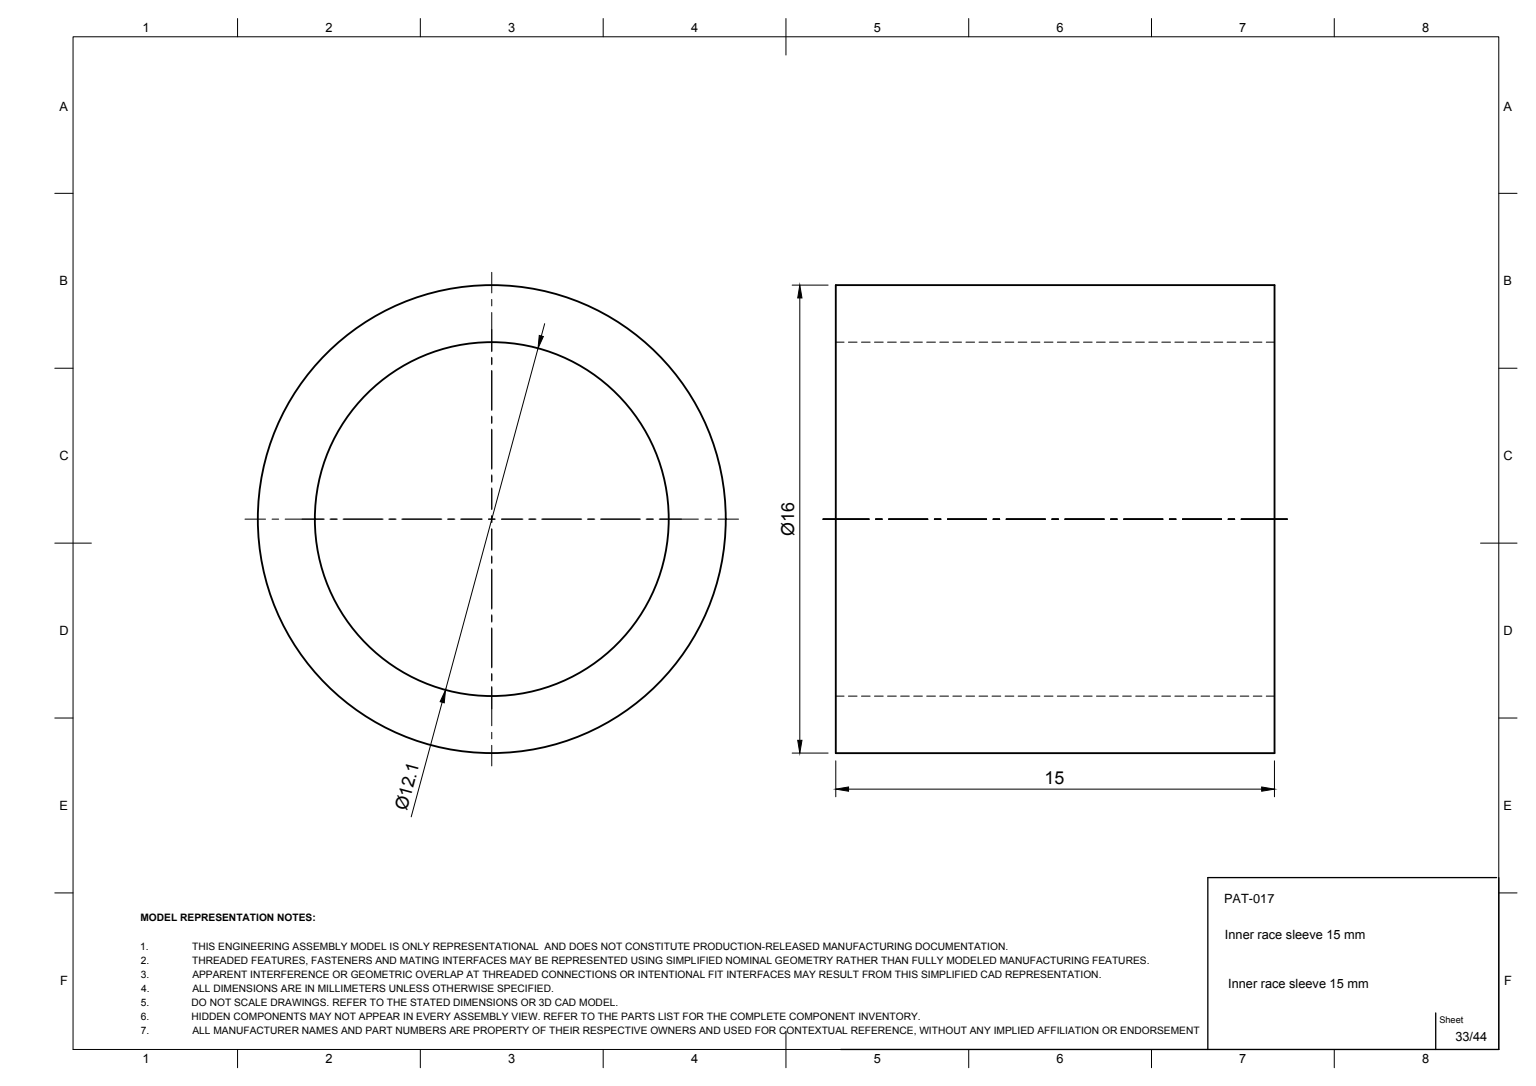
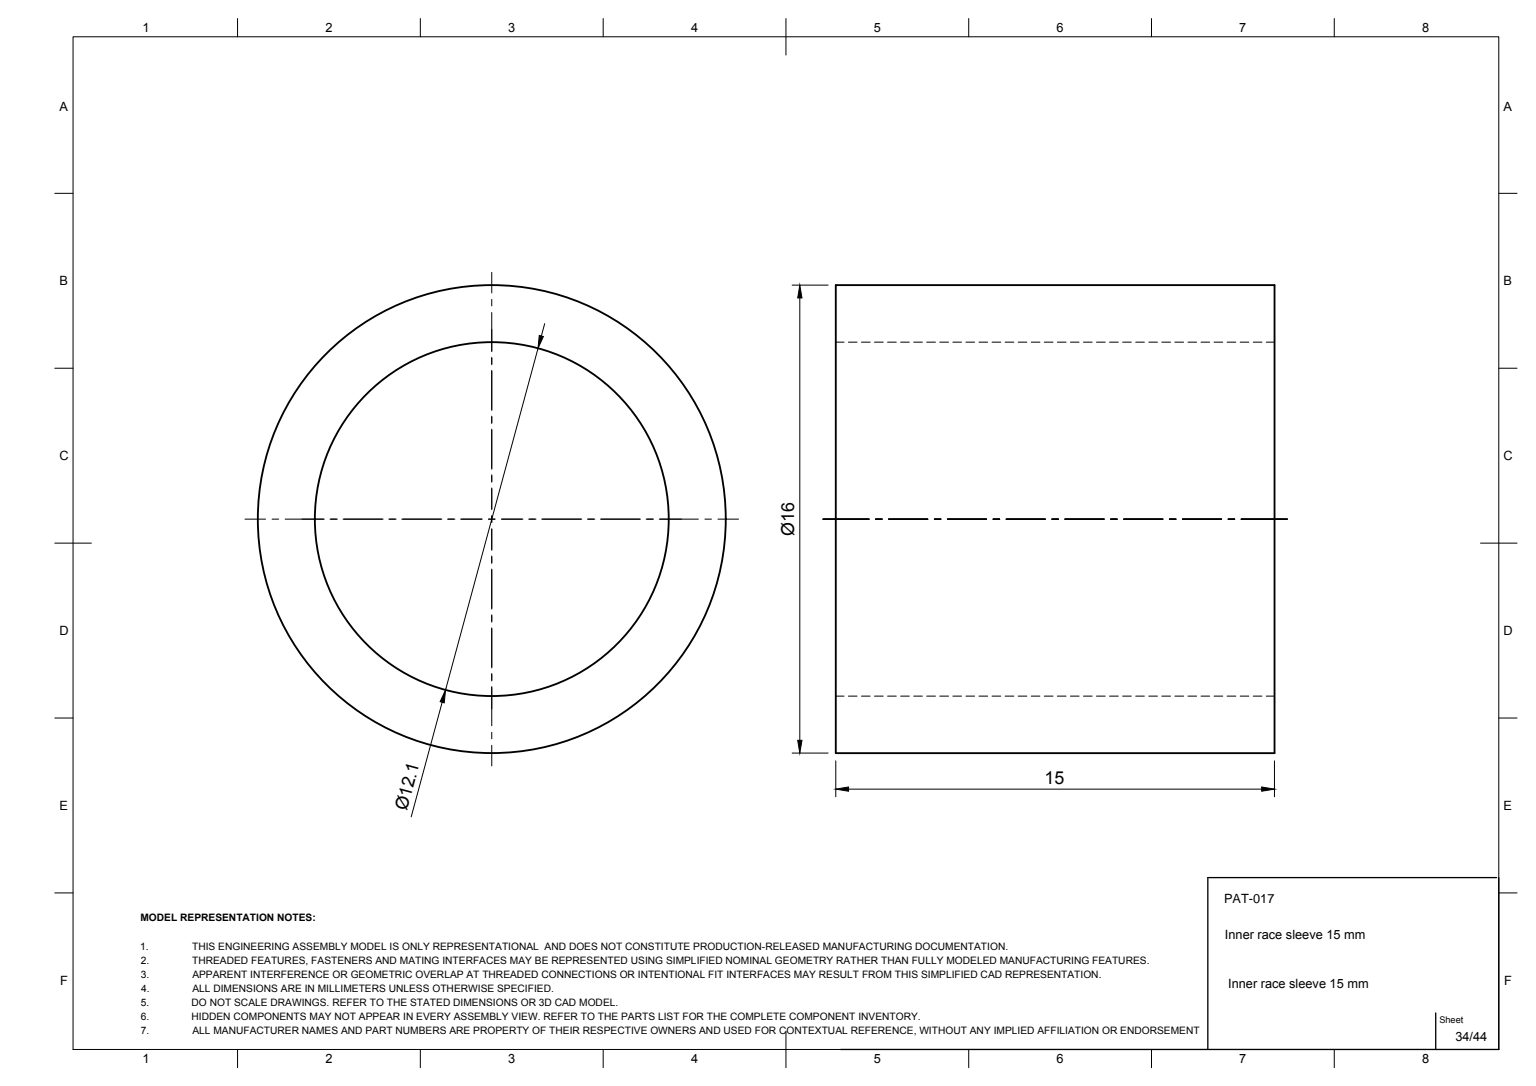
ISO-10303-21;
HEADER;
/* Generated by software containing ST-Developer
 * from STEP Tools, Inc. (www.steptools.com) 
 */

FILE_DESCRIPTION(
/* description */ ('Cam-and-follower valve demonstrator'),
/* implementation_level */ '2;1');

FILE_NAME(
/* name */ 'Inner race sleeve 15 mm.step',
/* time_stamp */ '2026-10-28T03:25:17-07:00',
/* author */ (''),
/* organization */ (''),
/* preprocessor_version */ 'ST-DEVELOPER v20.2',
/* originating_system */ 'Autodesk Translation Framework v15.17.0.0',
/* authorisation */ '');

FILE_SCHEMA (('AUTOMOTIVE_DESIGN { 1 0 10303 214 3 1 1 }'));
ENDSEC;

DATA;
#10=MECHANICAL_DESIGN_GEOMETRIC_PRESENTATION_REPRESENTATION('',(#443),#12896);
#364=SHAPE_REPRESENTATION_RELATIONSHIP('SRR','None',#13083,#400);
#400=ADVANCED_BREP_SHAPE_REPRESENTATION('',(#484),#12883);
#443=STYLED_ITEM('',(#13330),#484);
#484=MANIFOLD_SOLID_BREP('Body1',#6212);
#634=FACE_BOUND('',#1883,.T.);
#635=FACE_BOUND('',#1885,.T.);
#915=CIRCLE('',#7193,0.605);
#916=CIRCLE('',#7194,0.605);
#917=CIRCLE('',#7196,0.8);
#918=CIRCLE('',#7197,0.8);
#1069=CYLINDRICAL_SURFACE('',#7192,0.605);
#1070=CYLINDRICAL_SURFACE('',#7195,0.8);
#1373=FACE_OUTER_BOUND('',#1880,.T.);
#1374=FACE_OUTER_BOUND('',#1881,.T.);
#1375=FACE_OUTER_BOUND('',#1882,.T.);
#1376=FACE_OUTER_BOUND('',#1884,.T.);
#1880=EDGE_LOOP('',(#5263,#5264,#5265,#5266));
#1881=EDGE_LOOP('',(#5267,#5268,#5269,#5270));
#1882=EDGE_LOOP('',(#5271));
#1883=EDGE_LOOP('',(#5272));
#1884=EDGE_LOOP('',(#5273));
#1885=EDGE_LOOP('',(#5274));
#2308=LINE('',#12374,#2730);
#2309=LINE('',#12380,#2731);
#2730=VECTOR('',#8871,0.605);
#2731=VECTOR('',#8878,0.8);
#3234=VERTEX_POINT('',#12371);
#3235=VERTEX_POINT('',#12373);
#3236=VERTEX_POINT('',#12377);
#3237=VERTEX_POINT('',#12379);
#3928=EDGE_CURVE('',#3234,#3234,#915,.T.);
#3929=EDGE_CURVE('',#3234,#3235,#2308,.T.);
#3930=EDGE_CURVE('',#3235,#3235,#916,.T.);
#3931=EDGE_CURVE('',#3236,#3236,#917,.T.);
#3932=EDGE_CURVE('',#3236,#3237,#2309,.T.);
#3933=EDGE_CURVE('',#3237,#3237,#918,.T.);
#5263=ORIENTED_EDGE('',*,*,#3928,.F.);
#5264=ORIENTED_EDGE('',*,*,#3929,.T.);
#5265=ORIENTED_EDGE('',*,*,#3930,.T.);
#5266=ORIENTED_EDGE('',*,*,#3929,.F.);
#5267=ORIENTED_EDGE('',*,*,#3931,.F.);
#5268=ORIENTED_EDGE('',*,*,#3932,.T.);
#5269=ORIENTED_EDGE('',*,*,#3933,.T.);
#5270=ORIENTED_EDGE('',*,*,#3932,.F.);
#5271=ORIENTED_EDGE('',*,*,#3931,.T.);
#5272=ORIENTED_EDGE('',*,*,#3928,.T.);
#5273=ORIENTED_EDGE('',*,*,#3933,.F.);
#5274=ORIENTED_EDGE('',*,*,#3930,.F.);
#5751=PLANE('',#7198);
#5752=PLANE('',#7199);
#6089=ADVANCED_FACE('',(#1373),#1069,.F.);
#6090=ADVANCED_FACE('',(#1374),#1070,.T.);
#6091=ADVANCED_FACE('',(#1375,#634),#5751,.T.);
#6092=ADVANCED_FACE('',(#1376,#635),#5752,.F.);
#6212=CLOSED_SHELL('',(#6089,#6090,#6091,#6092));
#7191=AXIS2_PLACEMENT_3D('',#12369,#8865,#8866);
#7192=AXIS2_PLACEMENT_3D('',#12370,#8867,#8868);
#7193=AXIS2_PLACEMENT_3D('',#12372,#8869,#8870);
#7194=AXIS2_PLACEMENT_3D('',#12375,#8872,#8873);
#7195=AXIS2_PLACEMENT_3D('',#12376,#8874,#8875);
#7196=AXIS2_PLACEMENT_3D('',#12378,#8876,#8877);
#7197=AXIS2_PLACEMENT_3D('',#12381,#8879,#8880);
#7198=AXIS2_PLACEMENT_3D('',#12382,#8881,#8882);
#7199=AXIS2_PLACEMENT_3D('',#12383,#8883,#8884);
#8865=DIRECTION('axis',(0.,0.,1.));
#8866=DIRECTION('refdir',(1.,0.,0.));
#8867=DIRECTION('center_axis',(0.,1.,0.));
#8868=DIRECTION('ref_axis',(1.,0.,0.));
#8869=DIRECTION('center_axis',(0.,-1.,0.));
#8870=DIRECTION('ref_axis',(1.,0.,0.));
#8871=DIRECTION('',(0.,-1.,0.));
#8872=DIRECTION('center_axis',(0.,-1.,0.));
#8873=DIRECTION('ref_axis',(1.,0.,0.));
#8874=DIRECTION('center_axis',(0.,1.,0.));
#8875=DIRECTION('ref_axis',(1.,0.,0.));
#8876=DIRECTION('center_axis',(0.,1.,0.));
#8877=DIRECTION('ref_axis',(1.,0.,0.));
#8878=DIRECTION('',(0.,-1.,0.));
#8879=DIRECTION('center_axis',(0.,1.,0.));
#8880=DIRECTION('ref_axis',(1.,0.,0.));
#8881=DIRECTION('center_axis',(0.,1.,0.));
#8882=DIRECTION('ref_axis',(1.,0.,0.));
#8883=DIRECTION('center_axis',(0.,1.,0.));
#8884=DIRECTION('ref_axis',(1.,0.,0.));
#12369=CARTESIAN_POINT('',(0.,0.,0.));
#12370=CARTESIAN_POINT('Origin',(0.,-4.5,4.));
#12371=CARTESIAN_POINT('',(-0.605,-3.,4.));
#12372=CARTESIAN_POINT('Origin',(0.,-3.,4.));
#12373=CARTESIAN_POINT('',(-0.605,-4.5,4.));
#12374=CARTESIAN_POINT('',(-0.605,-4.5,4.));
#12375=CARTESIAN_POINT('Origin',(0.,-4.5,4.));
#12376=CARTESIAN_POINT('Origin',(0.,-4.5,4.));
#12377=CARTESIAN_POINT('',(-0.8,-3.,4.));
#12378=CARTESIAN_POINT('Origin',(0.,-3.,4.));
#12379=CARTESIAN_POINT('',(-0.8,-4.5,4.));
#12380=CARTESIAN_POINT('',(-0.8,-4.5,4.));
#12381=CARTESIAN_POINT('Origin',(0.,-4.5,4.));
#12382=CARTESIAN_POINT('Origin',(0.,-3.,4.));
#12383=CARTESIAN_POINT('Origin',(0.,-4.5,4.));
#12840=UNCERTAINTY_MEASURE_WITH_UNIT(LENGTH_MEASURE(0.001),#12897,
'DISTANCE_ACCURACY_VALUE',
'Maximum model space distance between geometric entities at asserted c
onnectivities');
#12853=UNCERTAINTY_MEASURE_WITH_UNIT(LENGTH_MEASURE(0.001),#12897,
'DISTANCE_ACCURACY_VALUE',
'Maximum model space distance between geometric entities at asserted c
onnectivities');
#12883=(
GEOMETRIC_REPRESENTATION_CONTEXT(3)
GLOBAL_UNCERTAINTY_ASSIGNED_CONTEXT((#12840))
GLOBAL_UNIT_ASSIGNED_CONTEXT((#12897,#12899,#12900))
REPRESENTATION_CONTEXT('','3D')
);
#12896=(
GEOMETRIC_REPRESENTATION_CONTEXT(3)
GLOBAL_UNCERTAINTY_ASSIGNED_CONTEXT((#12853))
GLOBAL_UNIT_ASSIGNED_CONTEXT((#12897,#12899,#12900))
REPRESENTATION_CONTEXT('','3D')
);
#12897=(
LENGTH_UNIT()
NAMED_UNIT(*)
SI_UNIT(.CENTI.,.METRE.)
);
#12899=(
NAMED_UNIT(*)
PLANE_ANGLE_UNIT()
SI_UNIT($,.RADIAN.)
);
#12900=(
NAMED_UNIT(*)
SI_UNIT($,.STERADIAN.)
SOLID_ANGLE_UNIT()
);
#12930=SHAPE_DEFINITION_REPRESENTATION(#12979,#13083);
#12979=PRODUCT_DEFINITION_SHAPE('',$,#13126);
#13083=SHAPE_REPRESENTATION('',(#7191),#12883);
#13096=PRODUCT_DEFINITION_CONTEXT('part definition',#13224,'design');
#13126=PRODUCT_DEFINITION('Inner race sleeve 15 mm',
'Inner race sleeve 15 mm',#13168,#13096);
#13168=PRODUCT_DEFINITION_FORMATION('',$,#13255);
#13224=APPLICATION_CONTEXT(
'Core Data for Automotive Mechanical Design Process');
#13225=PRODUCT_CONTEXT('part definition',#13224,'mechanical');
#13255=PRODUCT('Inner race sleeve 15 mm','Inner race sleeve 15 mm',
'Inner race sleeve 15 mm',(#13225));
#13324=COLOUR_RGB('Grey',0.48,0.52,0.57);
#13325=FILL_AREA_STYLE_COLOUR('',#13324);
#13326=FILL_AREA_STYLE('',(#13325));
#13327=SURFACE_STYLE_FILL_AREA(#13326);
#13328=SURFACE_SIDE_STYLE('',(#13327));
#13329=SURFACE_STYLE_USAGE(.BOTH.,#13328);
#13330=PRESENTATION_STYLE_ASSIGNMENT((#13329));
ENDSEC;
END-ISO-10303-21;
